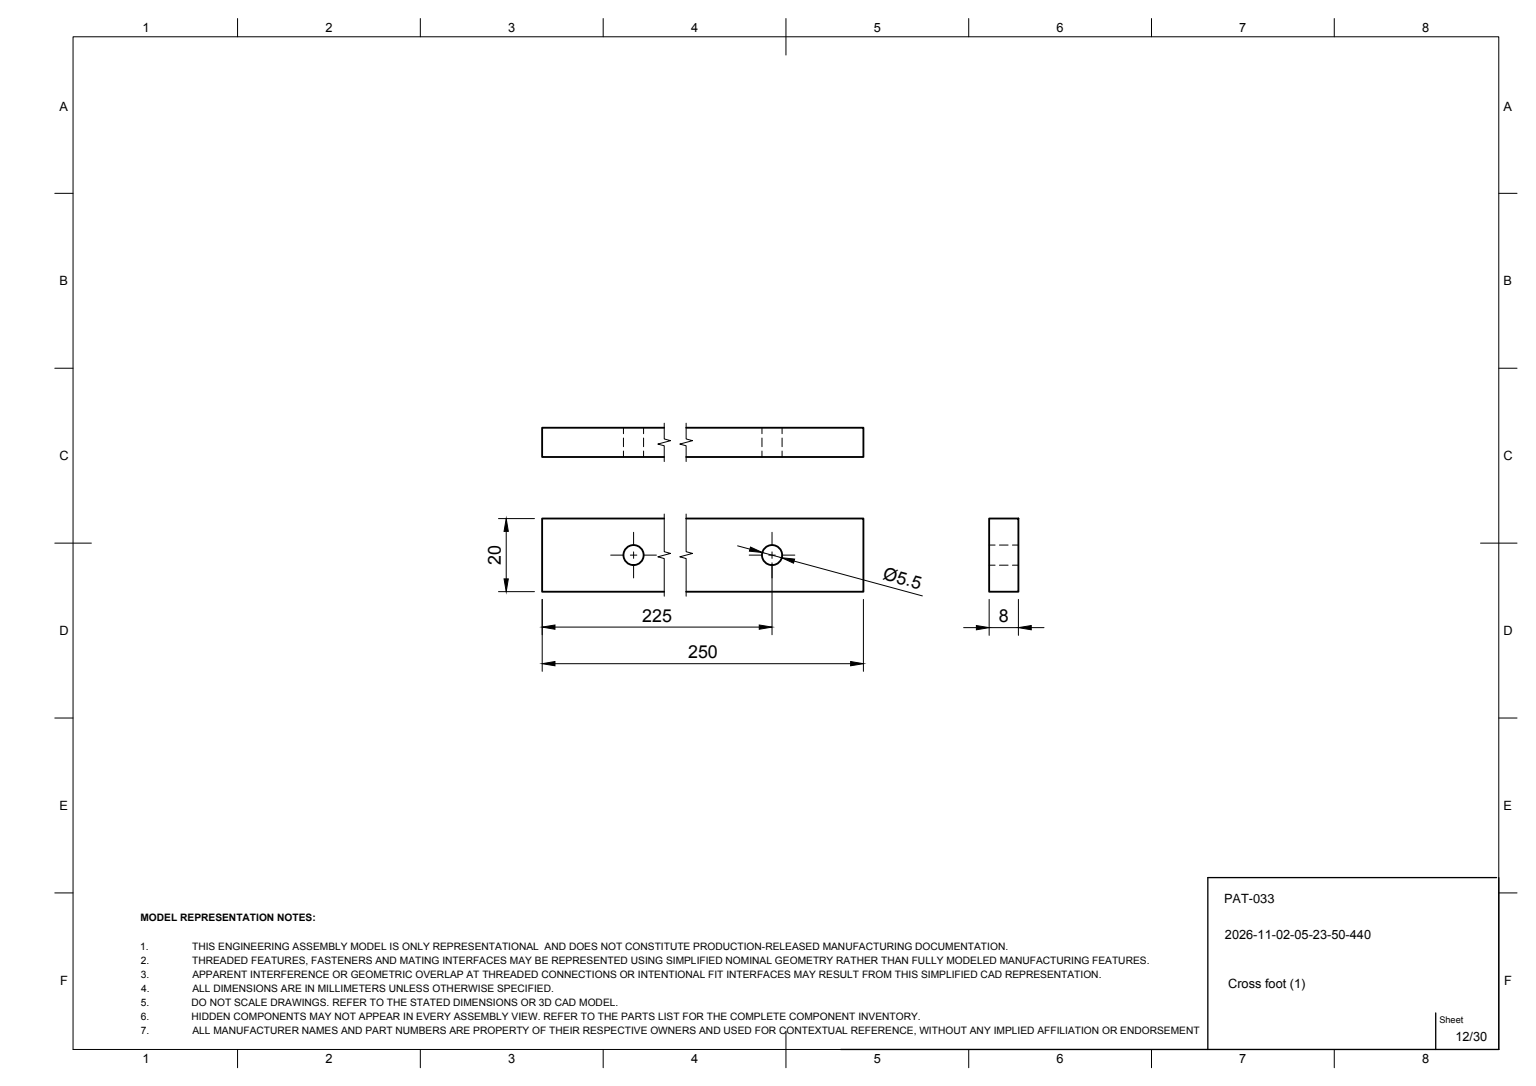
ISO-10303-21;
HEADER;
/* Generated by software containing ST-Developer
 * from STEP Tools, Inc. (www.steptools.com) 
 */

FILE_DESCRIPTION(
/* description */ ('Dual-rail gantry carriage'),
/* implementation_level */ '2;1');

FILE_NAME(
/* name */ 'Cross foot (1).step',
/* time_stamp */ '2026-10-27T10:49:15-07:00',
/* author */ (''),
/* organization */ (''),
/* preprocessor_version */ 'ST-DEVELOPER v20.2',
/* originating_system */ 'Autodesk Translation Framework v15.17.0.0',
/* authorisation */ '');

FILE_SCHEMA (('AUTOMOTIVE_DESIGN { 1 0 10303 214 3 1 1 }'));
ENDSEC;

DATA;
#10=MECHANICAL_DESIGN_GEOMETRIC_PRESENTATION_REPRESENTATION('',(#592),#12804);
#530=SHAPE_REPRESENTATION_RELATIONSHIP('SRR','None',#13008,#561);
#561=ADVANCED_BREP_SHAPE_REPRESENTATION('',(#623),#12778);
#592=STYLED_ITEM('',(#13261),#623);
#623=MANIFOLD_SOLID_BREP('Body1',#7370);
#678=FACE_BOUND('',#1540,.T.);
#679=FACE_BOUND('',#1541,.T.);
#680=FACE_BOUND('',#1543,.T.);
#681=FACE_BOUND('',#1544,.T.);
#806=PLANE('',#7853);
#807=PLANE('',#7854);
#808=PLANE('',#7855);
#809=PLANE('',#7856);
#810=PLANE('',#7857);
#811=PLANE('',#7858);
#1108=FACE_OUTER_BOUND('',#1533,.T.);
#1109=FACE_OUTER_BOUND('',#1534,.T.);
#1110=FACE_OUTER_BOUND('',#1535,.T.);
#1111=FACE_OUTER_BOUND('',#1536,.T.);
#1112=FACE_OUTER_BOUND('',#1537,.T.);
#1113=FACE_OUTER_BOUND('',#1538,.T.);
#1114=FACE_OUTER_BOUND('',#1539,.T.);
#1115=FACE_OUTER_BOUND('',#1542,.T.);
#1533=EDGE_LOOP('',(#5343,#5344,#5345,#5346));
#1534=EDGE_LOOP('',(#5347,#5348,#5349,#5350));
#1535=EDGE_LOOP('',(#5351,#5352,#5353,#5354));
#1536=EDGE_LOOP('',(#5355,#5356,#5357,#5358));
#1537=EDGE_LOOP('',(#5359,#5360,#5361,#5362));
#1538=EDGE_LOOP('',(#5363,#5364,#5365,#5366));
#1539=EDGE_LOOP('',(#5367,#5368,#5369,#5370));
#1540=EDGE_LOOP('',(#5371));
#1541=EDGE_LOOP('',(#5372));
#1542=EDGE_LOOP('',(#5373,#5374,#5375,#5376));
#1543=EDGE_LOOP('',(#5377));
#1544=EDGE_LOOP('',(#5378));
#2050=LINE('',#10992,#2759);
#2051=LINE('',#10998,#2760);
#2052=LINE('',#11003,#2761);
#2053=LINE('',#11005,#2762);
#2054=LINE('',#11007,#2763);
#2055=LINE('',#11008,#2764);
#2056=LINE('',#11011,#2765);
#2057=LINE('',#11013,#2766);
#2058=LINE('',#11014,#2767);
#2059=LINE('',#11017,#2768);
#2060=LINE('',#11019,#2769);
#2061=LINE('',#11020,#2770);
#2062=LINE('',#11022,#2771);
#2063=LINE('',#11023,#2772);
#2759=VECTOR('',#8805,0.274999999999999);
#2760=VECTOR('',#8812,0.274999999999999);
#2761=VECTOR('',#8817,1.);
#2762=VECTOR('',#8818,1.);
#2763=VECTOR('',#8819,1.);
#2764=VECTOR('',#8820,1.);
#2765=VECTOR('',#8823,1.);
#2766=VECTOR('',#8824,1.);
#2767=VECTOR('',#8825,1.);
#2768=VECTOR('',#8828,1.);
#2769=VECTOR('',#8829,1.);
#2770=VECTOR('',#8830,1.);
#2771=VECTOR('',#8833,1.);
#2772=VECTOR('',#8834,1.);
#3402=CIRCLE('',#7848,0.274999999999999);
#3403=CIRCLE('',#7849,0.274999999999999);
#3404=CIRCLE('',#7851,0.274999999999999);
#3405=CIRCLE('',#7852,0.274999999999999);
#3658=VERTEX_POINT('',#10989);
#3659=VERTEX_POINT('',#10991);
#3660=VERTEX_POINT('',#10995);
#3661=VERTEX_POINT('',#10997);
#3662=VERTEX_POINT('',#11001);
#3663=VERTEX_POINT('',#11002);
#3664=VERTEX_POINT('',#11004);
#3665=VERTEX_POINT('',#11006);
#3666=VERTEX_POINT('',#11010);
#3667=VERTEX_POINT('',#11012);
#3668=VERTEX_POINT('',#11016);
#3669=VERTEX_POINT('',#11018);
#4294=EDGE_CURVE('',#3658,#3658,#3402,.T.);
#4295=EDGE_CURVE('',#3658,#3659,#2050,.T.);
#4296=EDGE_CURVE('',#3659,#3659,#3403,.T.);
#4297=EDGE_CURVE('',#3660,#3660,#3404,.T.);
#4298=EDGE_CURVE('',#3660,#3661,#2051,.T.);
#4299=EDGE_CURVE('',#3661,#3661,#3405,.T.);
#4300=EDGE_CURVE('',#3662,#3663,#2052,.T.);
#4301=EDGE_CURVE('',#3663,#3664,#2053,.T.);
#4302=EDGE_CURVE('',#3665,#3664,#2054,.T.);
#4303=EDGE_CURVE('',#3662,#3665,#2055,.T.);
#4304=EDGE_CURVE('',#3666,#3662,#2056,.T.);
#4305=EDGE_CURVE('',#3667,#3665,#2057,.T.);
#4306=EDGE_CURVE('',#3666,#3667,#2058,.T.);
#4307=EDGE_CURVE('',#3668,#3666,#2059,.T.);
#4308=EDGE_CURVE('',#3669,#3667,#2060,.T.);
#4309=EDGE_CURVE('',#3668,#3669,#2061,.T.);
#4310=EDGE_CURVE('',#3663,#3668,#2062,.T.);
#4311=EDGE_CURVE('',#3664,#3669,#2063,.T.);
#5343=ORIENTED_EDGE('',*,*,#4294,.F.);
#5344=ORIENTED_EDGE('',*,*,#4295,.T.);
#5345=ORIENTED_EDGE('',*,*,#4296,.F.);
#5346=ORIENTED_EDGE('',*,*,#4295,.F.);
#5347=ORIENTED_EDGE('',*,*,#4297,.F.);
#5348=ORIENTED_EDGE('',*,*,#4298,.T.);
#5349=ORIENTED_EDGE('',*,*,#4299,.F.);
#5350=ORIENTED_EDGE('',*,*,#4298,.F.);
#5351=ORIENTED_EDGE('',*,*,#4300,.T.);
#5352=ORIENTED_EDGE('',*,*,#4301,.T.);
#5353=ORIENTED_EDGE('',*,*,#4302,.F.);
#5354=ORIENTED_EDGE('',*,*,#4303,.F.);
#5355=ORIENTED_EDGE('',*,*,#4304,.T.);
#5356=ORIENTED_EDGE('',*,*,#4303,.T.);
#5357=ORIENTED_EDGE('',*,*,#4305,.F.);
#5358=ORIENTED_EDGE('',*,*,#4306,.F.);
#5359=ORIENTED_EDGE('',*,*,#4307,.T.);
#5360=ORIENTED_EDGE('',*,*,#4306,.T.);
#5361=ORIENTED_EDGE('',*,*,#4308,.F.);
#5362=ORIENTED_EDGE('',*,*,#4309,.F.);
#5363=ORIENTED_EDGE('',*,*,#4310,.T.);
#5364=ORIENTED_EDGE('',*,*,#4309,.T.);
#5365=ORIENTED_EDGE('',*,*,#4311,.F.);
#5366=ORIENTED_EDGE('',*,*,#4301,.F.);
#5367=ORIENTED_EDGE('',*,*,#4311,.T.);
#5368=ORIENTED_EDGE('',*,*,#4308,.T.);
#5369=ORIENTED_EDGE('',*,*,#4305,.T.);
#5370=ORIENTED_EDGE('',*,*,#4302,.T.);
#5371=ORIENTED_EDGE('',*,*,#4296,.T.);
#5372=ORIENTED_EDGE('',*,*,#4299,.T.);
#5373=ORIENTED_EDGE('',*,*,#4310,.F.);
#5374=ORIENTED_EDGE('',*,*,#4300,.F.);
#5375=ORIENTED_EDGE('',*,*,#4304,.F.);
#5376=ORIENTED_EDGE('',*,*,#4307,.F.);
#5377=ORIENTED_EDGE('',*,*,#4294,.T.);
#5378=ORIENTED_EDGE('',*,*,#4297,.T.);
#6907=CYLINDRICAL_SURFACE('',#7847,0.274999999999999);
#6908=CYLINDRICAL_SURFACE('',#7850,0.274999999999999);
#7034=ADVANCED_FACE('',(#1108),#6907,.F.);
#7035=ADVANCED_FACE('',(#1109),#6908,.F.);
#7036=ADVANCED_FACE('',(#1110),#806,.T.);
#7037=ADVANCED_FACE('',(#1111),#807,.T.);
#7038=ADVANCED_FACE('',(#1112),#808,.T.);
#7039=ADVANCED_FACE('',(#1113),#809,.T.);
#7040=ADVANCED_FACE('',(#1114,#678,#679),#810,.T.);
#7041=ADVANCED_FACE('',(#1115,#680,#681),#811,.F.);
#7370=CLOSED_SHELL('',(#7034,#7035,#7036,#7037,#7038,#7039,#7040,#7041));
#7846=AXIS2_PLACEMENT_3D('',#10987,#8799,#8800);
#7847=AXIS2_PLACEMENT_3D('',#10988,#8801,#8802);
#7848=AXIS2_PLACEMENT_3D('',#10990,#8803,#8804);
#7849=AXIS2_PLACEMENT_3D('',#10993,#8806,#8807);
#7850=AXIS2_PLACEMENT_3D('',#10994,#8808,#8809);
#7851=AXIS2_PLACEMENT_3D('',#10996,#8810,#8811);
#7852=AXIS2_PLACEMENT_3D('',#10999,#8813,#8814);
#7853=AXIS2_PLACEMENT_3D('',#11000,#8815,#8816);
#7854=AXIS2_PLACEMENT_3D('',#11009,#8821,#8822);
#7855=AXIS2_PLACEMENT_3D('',#11015,#8826,#8827);
#7856=AXIS2_PLACEMENT_3D('',#11021,#8831,#8832);
#7857=AXIS2_PLACEMENT_3D('',#11024,#8835,#8836);
#7858=AXIS2_PLACEMENT_3D('',#11025,#8837,#8838);
#8799=DIRECTION('axis',(0.,0.,1.));
#8800=DIRECTION('refdir',(1.,0.,0.));
#8801=DIRECTION('center_axis',(0.,0.,1.));
#8802=DIRECTION('ref_axis',(1.,0.,0.));
#8803=DIRECTION('center_axis',(0.,0.,1.));
#8804=DIRECTION('ref_axis',(1.,0.,0.));
#8805=DIRECTION('',(0.,0.,1.));
#8806=DIRECTION('center_axis',(0.,0.,-1.));
#8807=DIRECTION('ref_axis',(1.,0.,0.));
#8808=DIRECTION('center_axis',(0.,0.,1.));
#8809=DIRECTION('ref_axis',(1.,0.,0.));
#8810=DIRECTION('center_axis',(0.,0.,1.));
#8811=DIRECTION('ref_axis',(1.,0.,0.));
#8812=DIRECTION('',(0.,0.,1.));
#8813=DIRECTION('center_axis',(0.,0.,-1.));
#8814=DIRECTION('ref_axis',(1.,0.,0.));
#8815=DIRECTION('center_axis',(0.,1.,0.));
#8816=DIRECTION('ref_axis',(-1.,0.,0.));
#8817=DIRECTION('',(-1.,0.,0.));
#8818=DIRECTION('',(0.,0.,1.));
#8819=DIRECTION('',(-1.,0.,0.));
#8820=DIRECTION('',(0.,0.,1.));
#8821=DIRECTION('center_axis',(1.,0.,0.));
#8822=DIRECTION('ref_axis',(0.,1.,0.));
#8823=DIRECTION('',(0.,1.,0.));
#8824=DIRECTION('',(0.,1.,0.));
#8825=DIRECTION('',(0.,0.,1.));
#8826=DIRECTION('center_axis',(0.,-1.,0.));
#8827=DIRECTION('ref_axis',(1.,0.,0.));
#8828=DIRECTION('',(1.,0.,0.));
#8829=DIRECTION('',(1.,0.,0.));
#8830=DIRECTION('',(0.,0.,1.));
#8831=DIRECTION('center_axis',(-1.,0.,0.));
#8832=DIRECTION('ref_axis',(0.,-1.,0.));
#8833=DIRECTION('',(0.,-1.,0.));
#8834=DIRECTION('',(0.,-1.,0.));
#8835=DIRECTION('center_axis',(0.,0.,1.));
#8836=DIRECTION('ref_axis',(1.,0.,0.));
#8837=DIRECTION('center_axis',(0.,0.,1.));
#8838=DIRECTION('ref_axis',(1.,0.,0.));
#10987=CARTESIAN_POINT('',(0.,0.,0.));
#10988=CARTESIAN_POINT('Origin',(39.,-10.,-0.9));
#10989=CARTESIAN_POINT('',(38.725,-10.,-0.8));
#10990=CARTESIAN_POINT('Origin',(39.,-10.,-0.8));
#10991=CARTESIAN_POINT('',(38.725,-10.,0.));
#10992=CARTESIAN_POINT('',(38.725,-10.,-0.9));
#10993=CARTESIAN_POINT('Origin',(39.,-10.,0.));
#10994=CARTESIAN_POINT('Origin',(39.,10.,-0.9));
#10995=CARTESIAN_POINT('',(38.725,10.,-0.8));
#10996=CARTESIAN_POINT('Origin',(39.,10.,-0.8));
#10997=CARTESIAN_POINT('',(38.725,10.,0.));
#10998=CARTESIAN_POINT('',(38.725,10.,-0.9));
#10999=CARTESIAN_POINT('Origin',(39.,10.,0.));
#11000=CARTESIAN_POINT('Origin',(40.,12.5,-0.8));
#11001=CARTESIAN_POINT('',(40.,12.5,-0.8));
#11002=CARTESIAN_POINT('',(38.,12.5,-0.8));
#11003=CARTESIAN_POINT('',(40.,12.5,-0.8));
#11004=CARTESIAN_POINT('',(38.,12.5,0.));
#11005=CARTESIAN_POINT('',(38.,12.5,-0.8));
#11006=CARTESIAN_POINT('',(40.,12.5,0.));
#11007=CARTESIAN_POINT('',(40.,12.5,0.));
#11008=CARTESIAN_POINT('',(40.,12.5,-0.8));
#11009=CARTESIAN_POINT('Origin',(40.,-12.5,-0.8));
#11010=CARTESIAN_POINT('',(40.,-12.5,-0.8));
#11011=CARTESIAN_POINT('',(40.,-12.5,-0.8));
#11012=CARTESIAN_POINT('',(40.,-12.5,0.));
#11013=CARTESIAN_POINT('',(40.,-12.5,0.));
#11014=CARTESIAN_POINT('',(40.,-12.5,-0.8));
#11015=CARTESIAN_POINT('Origin',(38.,-12.5,-0.8));
#11016=CARTESIAN_POINT('',(38.,-12.5,-0.8));
#11017=CARTESIAN_POINT('',(38.,-12.5,-0.8));
#11018=CARTESIAN_POINT('',(38.,-12.5,0.));
#11019=CARTESIAN_POINT('',(38.,-12.5,0.));
#11020=CARTESIAN_POINT('',(38.,-12.5,-0.8));
#11021=CARTESIAN_POINT('Origin',(38.,12.5,-0.8));
#11022=CARTESIAN_POINT('',(38.,12.5,-0.8));
#11023=CARTESIAN_POINT('',(38.,12.5,0.));
#11024=CARTESIAN_POINT('Origin',(39.,0.,0.));
#11025=CARTESIAN_POINT('Origin',(39.,0.,-0.8));
#12742=UNCERTAINTY_MEASURE_WITH_UNIT(LENGTH_MEASURE(0.001),#12805,
'DISTANCE_ACCURACY_VALUE',
'Maximum model space distance between geometric entities at asserted c
onnectivities');
#12768=UNCERTAINTY_MEASURE_WITH_UNIT(LENGTH_MEASURE(0.001),#12805,
'DISTANCE_ACCURACY_VALUE',
'Maximum model space distance between geometric entities at asserted c
onnectivities');
#12778=(
GEOMETRIC_REPRESENTATION_CONTEXT(3)
GLOBAL_UNCERTAINTY_ASSIGNED_CONTEXT((#12742))
GLOBAL_UNIT_ASSIGNED_CONTEXT((#12805,#12807,#12808))
REPRESENTATION_CONTEXT('','3D')
);
#12804=(
GEOMETRIC_REPRESENTATION_CONTEXT(3)
GLOBAL_UNCERTAINTY_ASSIGNED_CONTEXT((#12768))
GLOBAL_UNIT_ASSIGNED_CONTEXT((#12805,#12807,#12808))
REPRESENTATION_CONTEXT('','3D')
);
#12805=(
LENGTH_UNIT()
NAMED_UNIT(*)
SI_UNIT(.CENTI.,.METRE.)
);
#12807=(
NAMED_UNIT(*)
PLANE_ANGLE_UNIT()
SI_UNIT($,.RADIAN.)
);
#12808=(
NAMED_UNIT(*)
SI_UNIT($,.STERADIAN.)
SOLID_ANGLE_UNIT()
);
#12818=SHAPE_DEFINITION_REPRESENTATION(#12853,#13008);
#12853=PRODUCT_DEFINITION_SHAPE('',$,#13044);
#13008=SHAPE_REPRESENTATION('',(#7846),#12778);
#13034=PRODUCT_DEFINITION_CONTEXT('part definition',#13141,'design');
#13044=PRODUCT_DEFINITION('Cross foot (1)','Cross foot (1)',#13079,#13034);
#13079=PRODUCT_DEFINITION_FORMATION('',$,#13152);
#13141=APPLICATION_CONTEXT(
'Core Data for Automotive Mechanical Design Process');
#13142=PRODUCT_CONTEXT('part definition',#13141,'mechanical');
#13152=PRODUCT('Cross foot (1)','Cross foot (1)','Cross foot (1)',(#13142));
#13255=COLOUR_RGB('Off White',0.89,0.88,0.83);
#13256=FILL_AREA_STYLE_COLOUR('',#13255);
#13257=FILL_AREA_STYLE('',(#13256));
#13258=SURFACE_STYLE_FILL_AREA(#13257);
#13259=SURFACE_SIDE_STYLE('',(#13258));
#13260=SURFACE_STYLE_USAGE(.BOTH.,#13259);
#13261=PRESENTATION_STYLE_ASSIGNMENT((#13260));
ENDSEC;
END-ISO-10303-21;
